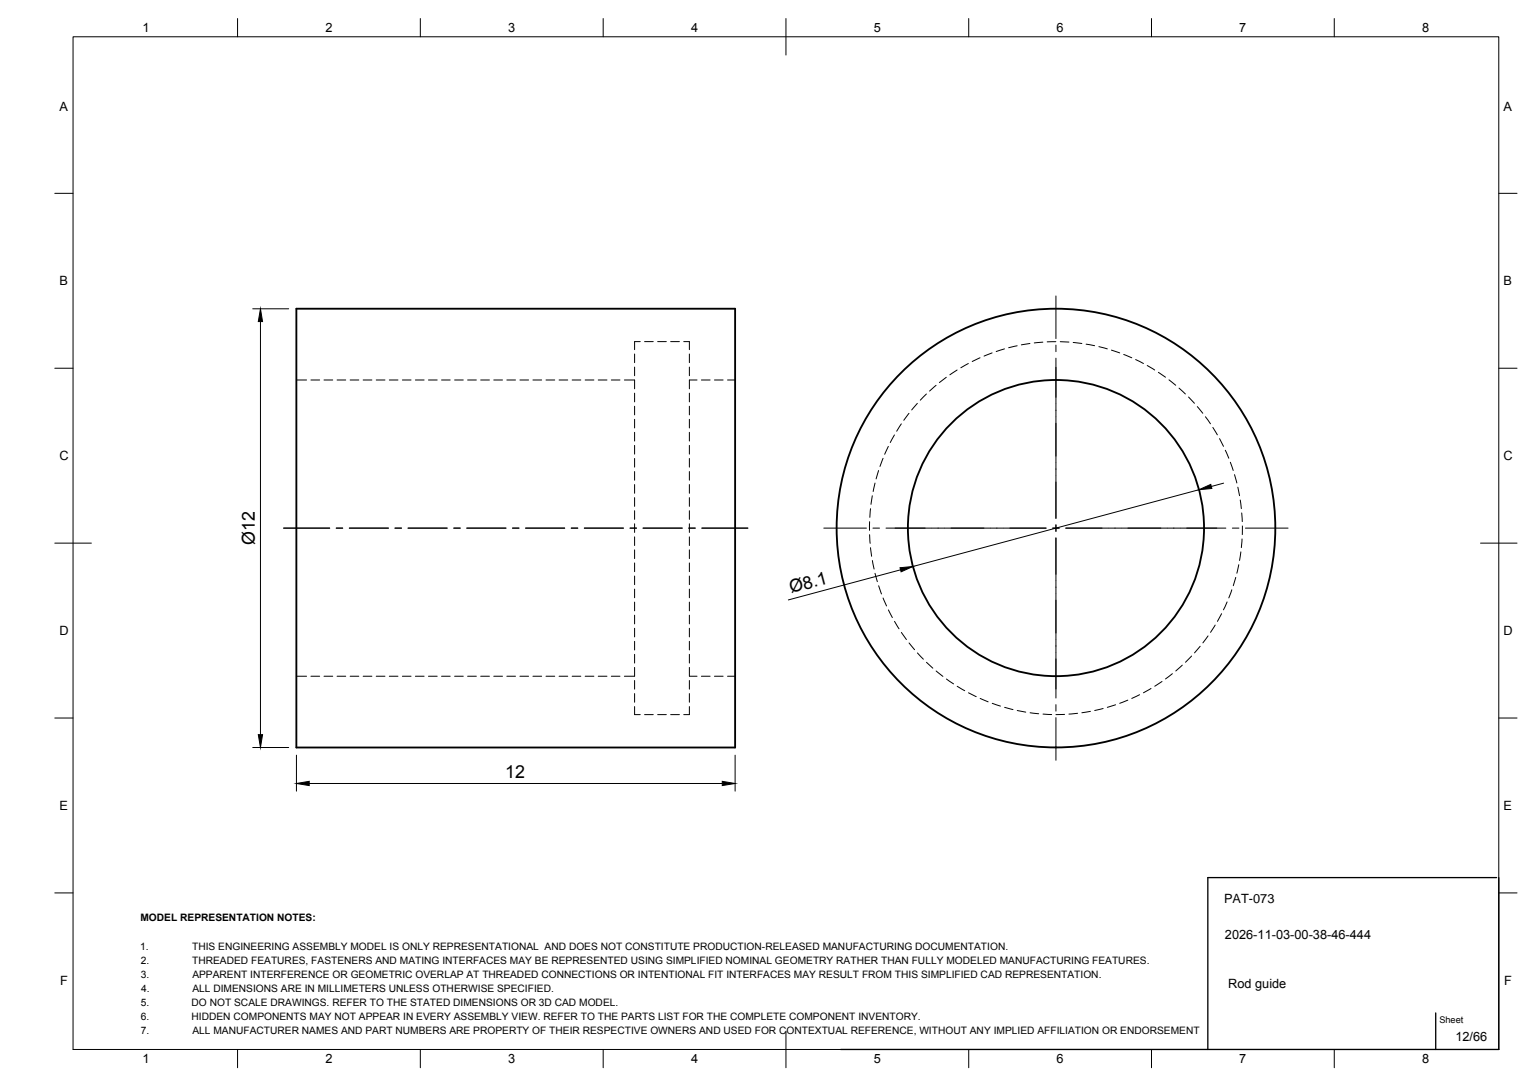
ISO-10303-21;
HEADER;
/* Generated by software containing ST-Developer
 * from STEP Tools, Inc. (www.steptools.com) 
 */

FILE_DESCRIPTION(
/* description */ ('Manual piston pump'),
/* implementation_level */ '2;1');

FILE_NAME(
/* name */ 'Rod guide.step',
/* time_stamp */ '2026-11-02T16:54:23-08:00',
/* author */ (''),
/* organization */ (''),
/* preprocessor_version */ 'ST-DEVELOPER v20.2',
/* originating_system */ 'Autodesk Translation Framework v15.17.0.0',
/* authorisation */ '');

FILE_SCHEMA (('AUTOMOTIVE_DESIGN { 1 0 10303 214 3 1 1 }'));
ENDSEC;

DATA;
#10=MECHANICAL_DESIGN_GEOMETRIC_PRESENTATION_REPRESENTATION('',(#695),#19043);
#569=SHAPE_REPRESENTATION_RELATIONSHIP('SRR','None',#19315,#632);
#632=ADVANCED_BREP_SHAPE_REPRESENTATION('',(#767),#18982);
#695=STYLED_ITEM('',(#19661),#767);
#767=MANIFOLD_SOLID_BREP('Body1',#9479);
#880=FACE_BOUND('',#2014,.T.);
#881=FACE_BOUND('',#2016,.T.);
#882=FACE_BOUND('',#2021,.T.);
#883=FACE_BOUND('',#2023,.T.);
#1134=CYLINDRICAL_SURFACE('',#10433,0.51);
#1135=CYLINDRICAL_SURFACE('',#10440,0.405);
#1136=CYLINDRICAL_SURFACE('',#10442,0.405);
#1137=CYLINDRICAL_SURFACE('',#10444,0.6);
#1384=FACE_OUTER_BOUND('',#2012,.T.);
#1385=FACE_OUTER_BOUND('',#2013,.T.);
#1386=FACE_OUTER_BOUND('',#2015,.T.);
#1387=FACE_OUTER_BOUND('',#2017,.T.);
#1388=FACE_OUTER_BOUND('',#2018,.T.);
#1389=FACE_OUTER_BOUND('',#2019,.T.);
#1390=FACE_OUTER_BOUND('',#2020,.T.);
#1391=FACE_OUTER_BOUND('',#2022,.T.);
#2012=EDGE_LOOP('',(#6683,#6684,#6685,#6686));
#2013=EDGE_LOOP('',(#6687));
#2014=EDGE_LOOP('',(#6688));
#2015=EDGE_LOOP('',(#6689));
#2016=EDGE_LOOP('',(#6690));
#2017=EDGE_LOOP('',(#6691,#6692,#6693,#6694));
#2018=EDGE_LOOP('',(#6695,#6696,#6697,#6698));
#2019=EDGE_LOOP('',(#6699,#6700,#6701,#6702));
#2020=EDGE_LOOP('',(#6703));
#2021=EDGE_LOOP('',(#6704));
#2022=EDGE_LOOP('',(#6705));
#2023=EDGE_LOOP('',(#6706));
#2751=CIRCLE('',#10434,0.51);
#2752=CIRCLE('',#10435,0.51);
#2753=CIRCLE('',#10437,0.405);
#2754=CIRCLE('',#10439,0.405);
#2755=CIRCLE('',#10441,0.405);
#2756=CIRCLE('',#10443,0.405);
#2757=CIRCLE('',#10445,0.6);
#2758=CIRCLE('',#10446,0.6);
#3261=LINE('',#15101,#3865);
#3262=LINE('',#15111,#3866);
#3263=LINE('',#15116,#3867);
#3264=LINE('',#15121,#3868);
#3865=VECTOR('',#11993,0.51);
#3866=VECTOR('',#12006,0.405);
#3867=VECTOR('',#12013,0.405);
#3868=VECTOR('',#12018,0.6);
#4491=VERTEX_POINT('',#15098);
#4492=VERTEX_POINT('',#15100);
#4493=VERTEX_POINT('',#15104);
#4494=VERTEX_POINT('',#15107);
#4495=VERTEX_POINT('',#15110);
#4496=VERTEX_POINT('',#15114);
#4497=VERTEX_POINT('',#15118);
#4498=VERTEX_POINT('',#15120);
#5328=EDGE_CURVE('',#4491,#4491,#2751,.T.);
#5329=EDGE_CURVE('',#4491,#4492,#3261,.T.);
#5330=EDGE_CURVE('',#4492,#4492,#2752,.T.);
#5331=EDGE_CURVE('',#4493,#4493,#2753,.T.);
#5332=EDGE_CURVE('',#4494,#4494,#2754,.T.);
#5333=EDGE_CURVE('',#4494,#4495,#3262,.T.);
#5334=EDGE_CURVE('',#4495,#4495,#2755,.T.);
#5335=EDGE_CURVE('',#4496,#4496,#2756,.T.);
#5336=EDGE_CURVE('',#4496,#4493,#3263,.T.);
#5337=EDGE_CURVE('',#4497,#4497,#2757,.T.);
#5338=EDGE_CURVE('',#4497,#4498,#3264,.T.);
#5339=EDGE_CURVE('',#4498,#4498,#2758,.T.);
#6683=ORIENTED_EDGE('',*,*,#5328,.F.);
#6684=ORIENTED_EDGE('',*,*,#5329,.T.);
#6685=ORIENTED_EDGE('',*,*,#5330,.T.);
#6686=ORIENTED_EDGE('',*,*,#5329,.F.);
#6687=ORIENTED_EDGE('',*,*,#5330,.F.);
#6688=ORIENTED_EDGE('',*,*,#5331,.F.);
#6689=ORIENTED_EDGE('',*,*,#5328,.T.);
#6690=ORIENTED_EDGE('',*,*,#5332,.F.);
#6691=ORIENTED_EDGE('',*,*,#5332,.T.);
#6692=ORIENTED_EDGE('',*,*,#5333,.T.);
#6693=ORIENTED_EDGE('',*,*,#5334,.T.);
#6694=ORIENTED_EDGE('',*,*,#5333,.F.);
#6695=ORIENTED_EDGE('',*,*,#5335,.F.);
#6696=ORIENTED_EDGE('',*,*,#5336,.T.);
#6697=ORIENTED_EDGE('',*,*,#5331,.T.);
#6698=ORIENTED_EDGE('',*,*,#5336,.F.);
#6699=ORIENTED_EDGE('',*,*,#5337,.F.);
#6700=ORIENTED_EDGE('',*,*,#5338,.T.);
#6701=ORIENTED_EDGE('',*,*,#5339,.T.);
#6702=ORIENTED_EDGE('',*,*,#5338,.F.);
#6703=ORIENTED_EDGE('',*,*,#5337,.T.);
#6704=ORIENTED_EDGE('',*,*,#5335,.T.);
#6705=ORIENTED_EDGE('',*,*,#5339,.F.);
#6706=ORIENTED_EDGE('',*,*,#5334,.F.);
#8622=PLANE('',#10436);
#8623=PLANE('',#10438);
#8624=PLANE('',#10447);
#8625=PLANE('',#10448);
#8989=ADVANCED_FACE('',(#1384),#1134,.F.);
#8990=ADVANCED_FACE('',(#1385,#880),#8622,.F.);
#8991=ADVANCED_FACE('',(#1386,#881),#8623,.T.);
#8992=ADVANCED_FACE('',(#1387),#1135,.F.);
#8993=ADVANCED_FACE('',(#1388),#1136,.F.);
#8994=ADVANCED_FACE('',(#1389),#1137,.T.);
#8995=ADVANCED_FACE('',(#1390,#882),#8624,.T.);
#8996=ADVANCED_FACE('',(#1391,#883),#8625,.F.);
#9479=CLOSED_SHELL('',(#8989,#8990,#8991,#8992,#8993,#8994,#8995,#8996));
#10432=AXIS2_PLACEMENT_3D('',#15096,#11987,#11988);
#10433=AXIS2_PLACEMENT_3D('',#15097,#11989,#11990);
#10434=AXIS2_PLACEMENT_3D('',#15099,#11991,#11992);
#10435=AXIS2_PLACEMENT_3D('',#15102,#11994,#11995);
#10436=AXIS2_PLACEMENT_3D('',#15103,#11996,#11997);
#10437=AXIS2_PLACEMENT_3D('',#15105,#11998,#11999);
#10438=AXIS2_PLACEMENT_3D('',#15106,#12000,#12001);
#10439=AXIS2_PLACEMENT_3D('',#15108,#12002,#12003);
#10440=AXIS2_PLACEMENT_3D('',#15109,#12004,#12005);
#10441=AXIS2_PLACEMENT_3D('',#15112,#12007,#12008);
#10442=AXIS2_PLACEMENT_3D('',#15113,#12009,#12010);
#10443=AXIS2_PLACEMENT_3D('',#15115,#12011,#12012);
#10444=AXIS2_PLACEMENT_3D('',#15117,#12014,#12015);
#10445=AXIS2_PLACEMENT_3D('',#15119,#12016,#12017);
#10446=AXIS2_PLACEMENT_3D('',#15122,#12019,#12020);
#10447=AXIS2_PLACEMENT_3D('',#15123,#12021,#12022);
#10448=AXIS2_PLACEMENT_3D('',#15124,#12023,#12024);
#11987=DIRECTION('axis',(0.,0.,1.));
#11988=DIRECTION('refdir',(1.,0.,0.));
#11989=DIRECTION('center_axis',(0.,1.,0.));
#11990=DIRECTION('ref_axis',(1.,0.,0.));
#11991=DIRECTION('center_axis',(0.,1.,0.));
#11992=DIRECTION('ref_axis',(1.,0.,0.));
#11993=DIRECTION('',(0.,1.,0.));
#11994=DIRECTION('center_axis',(0.,1.,0.));
#11995=DIRECTION('ref_axis',(1.,0.,0.));
#11996=DIRECTION('center_axis',(0.,1.,0.));
#11997=DIRECTION('ref_axis',(1.,0.,0.));
#11998=DIRECTION('center_axis',(0.,-1.,0.));
#11999=DIRECTION('ref_axis',(1.,0.,0.));
#12000=DIRECTION('center_axis',(0.,1.,0.));
#12001=DIRECTION('ref_axis',(1.,0.,0.));
#12002=DIRECTION('center_axis',(0.,1.,0.));
#12003=DIRECTION('ref_axis',(1.,0.,0.));
#12004=DIRECTION('center_axis',(0.,1.,0.));
#12005=DIRECTION('ref_axis',(1.,0.,0.));
#12006=DIRECTION('',(0.,-1.,0.));
#12007=DIRECTION('center_axis',(0.,-1.,0.));
#12008=DIRECTION('ref_axis',(1.,0.,0.));
#12009=DIRECTION('center_axis',(0.,1.,0.));
#12010=DIRECTION('ref_axis',(1.,0.,0.));
#12011=DIRECTION('center_axis',(0.,-1.,0.));
#12012=DIRECTION('ref_axis',(1.,0.,0.));
#12013=DIRECTION('',(0.,-1.,0.));
#12014=DIRECTION('center_axis',(0.,1.,0.));
#12015=DIRECTION('ref_axis',(1.,0.,0.));
#12016=DIRECTION('center_axis',(0.,1.,0.));
#12017=DIRECTION('ref_axis',(1.,0.,0.));
#12018=DIRECTION('',(0.,-1.,0.));
#12019=DIRECTION('center_axis',(0.,1.,0.));
#12020=DIRECTION('ref_axis',(1.,0.,0.));
#12021=DIRECTION('center_axis',(0.,1.,0.));
#12022=DIRECTION('ref_axis',(1.,0.,0.));
#12023=DIRECTION('center_axis',(0.,1.,0.));
#12024=DIRECTION('ref_axis',(1.,0.,0.));
#15096=CARTESIAN_POINT('',(0.,0.,0.));
#15097=CARTESIAN_POINT('Origin',(0.,0.125,4.5));
#15098=CARTESIAN_POINT('',(-0.51,0.125,4.5));
#15099=CARTESIAN_POINT('Origin',(0.,0.125,4.5));
#15100=CARTESIAN_POINT('',(-0.51,0.275,4.5));
#15101=CARTESIAN_POINT('',(-0.51,0.125,4.5));
#15102=CARTESIAN_POINT('Origin',(0.,0.275,4.5));
#15103=CARTESIAN_POINT('Origin',(0.,0.275,4.5));
#15104=CARTESIAN_POINT('',(-0.405,0.275,4.5));
#15105=CARTESIAN_POINT('Origin',(0.,0.275,4.5));
#15106=CARTESIAN_POINT('Origin',(0.,0.125,4.5));
#15107=CARTESIAN_POINT('',(-0.405,0.125,4.5));
#15108=CARTESIAN_POINT('Origin',(0.,0.125,4.5));
#15109=CARTESIAN_POINT('Origin',(0.,0.,4.5));
#15110=CARTESIAN_POINT('',(-0.405,0.,4.5));
#15111=CARTESIAN_POINT('',(-0.405,0.,4.5));
#15112=CARTESIAN_POINT('Origin',(0.,0.,4.5));
#15113=CARTESIAN_POINT('Origin',(0.,0.,4.5));
#15114=CARTESIAN_POINT('',(-0.405,1.2,4.5));
#15115=CARTESIAN_POINT('Origin',(0.,1.2,4.5));
#15116=CARTESIAN_POINT('',(-0.405,0.,4.5));
#15117=CARTESIAN_POINT('Origin',(0.,0.,4.5));
#15118=CARTESIAN_POINT('',(-0.6,1.2,4.5));
#15119=CARTESIAN_POINT('Origin',(0.,1.2,4.5));
#15120=CARTESIAN_POINT('',(-0.6,0.,4.5));
#15121=CARTESIAN_POINT('',(-0.6,0.,4.5));
#15122=CARTESIAN_POINT('Origin',(0.,0.,4.5));
#15123=CARTESIAN_POINT('Origin',(0.,1.2,4.5));
#15124=CARTESIAN_POINT('Origin',(0.,0.,4.5));
#18911=UNCERTAINTY_MEASURE_WITH_UNIT(LENGTH_MEASURE(0.001),#19044,
'DISTANCE_ACCURACY_VALUE',
'Maximum model space distance between geometric entities at asserted c
onnectivities');
#18972=UNCERTAINTY_MEASURE_WITH_UNIT(LENGTH_MEASURE(0.001),#19044,
'DISTANCE_ACCURACY_VALUE',
'Maximum model space distance between geometric entities at asserted c
onnectivities');
#18982=(
GEOMETRIC_REPRESENTATION_CONTEXT(3)
GLOBAL_UNCERTAINTY_ASSIGNED_CONTEXT((#18911))
GLOBAL_UNIT_ASSIGNED_CONTEXT((#19044,#19046,#19047))
REPRESENTATION_CONTEXT('','3D')
);
#19043=(
GEOMETRIC_REPRESENTATION_CONTEXT(3)
GLOBAL_UNCERTAINTY_ASSIGNED_CONTEXT((#18972))
GLOBAL_UNIT_ASSIGNED_CONTEXT((#19044,#19046,#19047))
REPRESENTATION_CONTEXT('','3D')
);
#19044=(
LENGTH_UNIT()
NAMED_UNIT(*)
SI_UNIT(.CENTI.,.METRE.)
);
#19046=(
NAMED_UNIT(*)
PLANE_ANGLE_UNIT()
SI_UNIT($,.RADIAN.)
);
#19047=(
NAMED_UNIT(*)
SI_UNIT($,.STERADIAN.)
SOLID_ANGLE_UNIT()
);
#19057=SHAPE_DEFINITION_REPRESENTATION(#19127,#19315);
#19127=PRODUCT_DEFINITION_SHAPE('',$,#19386);
#19315=SHAPE_REPRESENTATION('',(#10432),#18982);
#19376=PRODUCT_DEFINITION_CONTEXT('part definition',#19588,'design');
#19386=PRODUCT_DEFINITION('2026-11-03-00-38-46-444','Rod guide',#19456,
#19376);
#19456=PRODUCT_DEFINITION_FORMATION('',$,#19599);
#19588=APPLICATION_CONTEXT(
'Core Data for Automotive Mechanical Design Process');
#19589=PRODUCT_CONTEXT('part definition',#19588,'mechanical');
#19599=PRODUCT('2026-11-03-00-38-46-444','Rod guide','Rod guide',(#19589));
#19661=PRESENTATION_STYLE_ASSIGNMENT((#19667));
#19667=SURFACE_STYLE_USAGE(.BOTH.,#19673);
#19673=SURFACE_SIDE_STYLE('',(#19679));
#19679=SURFACE_STYLE_FILL_AREA(#19685);
#19685=FILL_AREA_STYLE('CAD Library Painted - Engineering blue',(#19691));
#19691=FILL_AREA_STYLE_COLOUR('CAD Library Painted - Engineering blue',
#19697);
#19697=COLOUR_RGB('CAD Library Painted - Engineering blue',0.12156862745098,
0.356862745098039,0.6);
ENDSEC;
END-ISO-10303-21;
